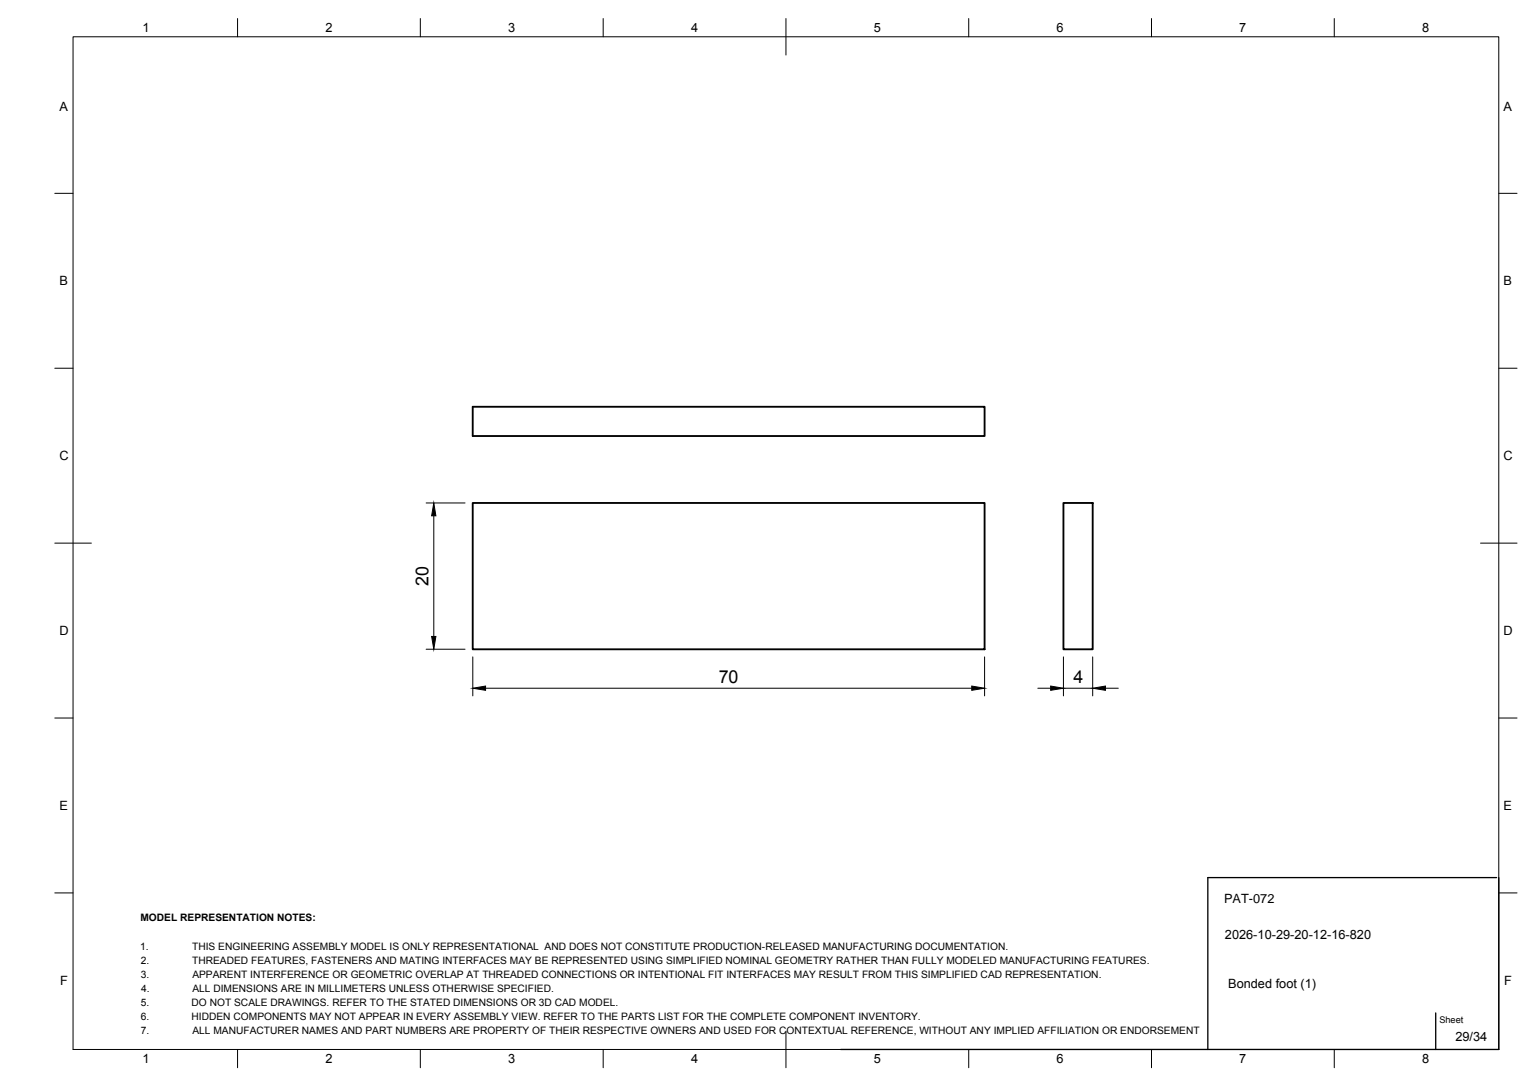
ISO-10303-21;
HEADER;
/* Generated by software containing ST-Developer
 * from STEP Tools, Inc. (www.steptools.com) 
 */

FILE_DESCRIPTION(
/* description */ ('PAT-072'),
/* implementation_level */ '2;1');

FILE_NAME(
/* name */ 'Bonded foot (1).step',
/* time_stamp */ '2026-10-29T20:11:56-07:00',
/* author */ (''),
/* organization */ (''),
/* preprocessor_version */ 'ST-DEVELOPER v20.2',
/* originating_system */ 'Autodesk Translation Framework v15.17.0.0',
/* authorisation */ '');

FILE_SCHEMA (('AUTOMOTIVE_DESIGN { 1 0 10303 214 3 1 1 }'));
ENDSEC;

DATA;
#10=MECHANICAL_DESIGN_GEOMETRIC_PRESENTATION_REPRESENTATION('',(#362),#11432);
#290=SHAPE_REPRESENTATION_RELATIONSHIP('SRR','None',#11594,#326);
#326=ADVANCED_BREP_SHAPE_REPRESENTATION('',(#398),#11425);
#362=STYLED_ITEM('',(#11833),#398);
#398=MANIFOLD_SOLID_BREP('Body1',#6097);
#743=PLANE('',#7087);
#744=PLANE('',#7088);
#745=PLANE('',#7089);
#746=PLANE('',#7090);
#747=PLANE('',#7091);
#748=PLANE('',#7092);
#1091=FACE_OUTER_BOUND('',#1616,.T.);
#1092=FACE_OUTER_BOUND('',#1617,.T.);
#1093=FACE_OUTER_BOUND('',#1618,.T.);
#1094=FACE_OUTER_BOUND('',#1619,.T.);
#1095=FACE_OUTER_BOUND('',#1620,.T.);
#1096=FACE_OUTER_BOUND('',#1621,.T.);
#1616=EDGE_LOOP('',(#5264,#5265,#5266,#5267));
#1617=EDGE_LOOP('',(#5268,#5269,#5270,#5271));
#1618=EDGE_LOOP('',(#5272,#5273,#5274,#5275));
#1619=EDGE_LOOP('',(#5276,#5277,#5278,#5279));
#1620=EDGE_LOOP('',(#5280,#5281,#5282,#5283));
#1621=EDGE_LOOP('',(#5284,#5285,#5286,#5287));
#2019=LINE('',#10983,#2438);
#2020=LINE('',#10985,#2439);
#2021=LINE('',#10987,#2440);
#2022=LINE('',#10988,#2441);
#2023=LINE('',#10991,#2442);
#2024=LINE('',#10993,#2443);
#2025=LINE('',#10994,#2444);
#2026=LINE('',#10997,#2445);
#2027=LINE('',#10999,#2446);
#2028=LINE('',#11000,#2447);
#2029=LINE('',#11002,#2448);
#2030=LINE('',#11003,#2449);
#2438=VECTOR('',#8742,1.);
#2439=VECTOR('',#8743,1.);
#2440=VECTOR('',#8744,1.);
#2441=VECTOR('',#8745,1.);
#2442=VECTOR('',#8748,1.);
#2443=VECTOR('',#8749,1.);
#2444=VECTOR('',#8750,1.);
#2445=VECTOR('',#8753,1.);
#2446=VECTOR('',#8754,1.);
#2447=VECTOR('',#8755,1.);
#2448=VECTOR('',#8758,1.);
#2449=VECTOR('',#8759,1.);
#3228=VERTEX_POINT('',#10981);
#3229=VERTEX_POINT('',#10982);
#3230=VERTEX_POINT('',#10984);
#3231=VERTEX_POINT('',#10986);
#3232=VERTEX_POINT('',#10990);
#3233=VERTEX_POINT('',#10992);
#3234=VERTEX_POINT('',#10996);
#3235=VERTEX_POINT('',#10998);
#3921=EDGE_CURVE('',#3228,#3229,#2019,.T.);
#3922=EDGE_CURVE('',#3229,#3230,#2020,.T.);
#3923=EDGE_CURVE('',#3231,#3230,#2021,.T.);
#3924=EDGE_CURVE('',#3228,#3231,#2022,.T.);
#3925=EDGE_CURVE('',#3232,#3228,#2023,.T.);
#3926=EDGE_CURVE('',#3233,#3231,#2024,.T.);
#3927=EDGE_CURVE('',#3232,#3233,#2025,.T.);
#3928=EDGE_CURVE('',#3234,#3232,#2026,.T.);
#3929=EDGE_CURVE('',#3235,#3233,#2027,.T.);
#3930=EDGE_CURVE('',#3234,#3235,#2028,.T.);
#3931=EDGE_CURVE('',#3229,#3234,#2029,.T.);
#3932=EDGE_CURVE('',#3230,#3235,#2030,.T.);
#5264=ORIENTED_EDGE('',*,*,#3921,.T.);
#5265=ORIENTED_EDGE('',*,*,#3922,.T.);
#5266=ORIENTED_EDGE('',*,*,#3923,.F.);
#5267=ORIENTED_EDGE('',*,*,#3924,.F.);
#5268=ORIENTED_EDGE('',*,*,#3925,.T.);
#5269=ORIENTED_EDGE('',*,*,#3924,.T.);
#5270=ORIENTED_EDGE('',*,*,#3926,.F.);
#5271=ORIENTED_EDGE('',*,*,#3927,.F.);
#5272=ORIENTED_EDGE('',*,*,#3928,.T.);
#5273=ORIENTED_EDGE('',*,*,#3927,.T.);
#5274=ORIENTED_EDGE('',*,*,#3929,.F.);
#5275=ORIENTED_EDGE('',*,*,#3930,.F.);
#5276=ORIENTED_EDGE('',*,*,#3931,.T.);
#5277=ORIENTED_EDGE('',*,*,#3930,.T.);
#5278=ORIENTED_EDGE('',*,*,#3932,.F.);
#5279=ORIENTED_EDGE('',*,*,#3922,.F.);
#5280=ORIENTED_EDGE('',*,*,#3932,.T.);
#5281=ORIENTED_EDGE('',*,*,#3929,.T.);
#5282=ORIENTED_EDGE('',*,*,#3926,.T.);
#5283=ORIENTED_EDGE('',*,*,#3923,.T.);
#5284=ORIENTED_EDGE('',*,*,#3931,.F.);
#5285=ORIENTED_EDGE('',*,*,#3921,.F.);
#5286=ORIENTED_EDGE('',*,*,#3925,.F.);
#5287=ORIENTED_EDGE('',*,*,#3928,.F.);
#5990=ADVANCED_FACE('',(#1091),#743,.T.);
#5991=ADVANCED_FACE('',(#1092),#744,.T.);
#5992=ADVANCED_FACE('',(#1093),#745,.T.);
#5993=ADVANCED_FACE('',(#1094),#746,.T.);
#5994=ADVANCED_FACE('',(#1095),#747,.T.);
#5995=ADVANCED_FACE('',(#1096),#748,.F.);
#6097=CLOSED_SHELL('',(#5990,#5991,#5992,#5993,#5994,#5995));
#7086=AXIS2_PLACEMENT_3D('',#10979,#8738,#8739);
#7087=AXIS2_PLACEMENT_3D('',#10980,#8740,#8741);
#7088=AXIS2_PLACEMENT_3D('',#10989,#8746,#8747);
#7089=AXIS2_PLACEMENT_3D('',#10995,#8751,#8752);
#7090=AXIS2_PLACEMENT_3D('',#11001,#8756,#8757);
#7091=AXIS2_PLACEMENT_3D('',#11004,#8760,#8761);
#7092=AXIS2_PLACEMENT_3D('',#11005,#8762,#8763);
#8738=DIRECTION('axis',(0.,0.,1.));
#8739=DIRECTION('refdir',(1.,0.,0.));
#8740=DIRECTION('center_axis',(0.,1.,0.));
#8741=DIRECTION('ref_axis',(-1.,0.,0.));
#8742=DIRECTION('',(-1.,0.,0.));
#8743=DIRECTION('',(0.,0.,1.));
#8744=DIRECTION('',(-1.,0.,0.));
#8745=DIRECTION('',(0.,0.,1.));
#8746=DIRECTION('center_axis',(1.,0.,0.));
#8747=DIRECTION('ref_axis',(0.,1.,0.));
#8748=DIRECTION('',(0.,1.,0.));
#8749=DIRECTION('',(0.,1.,0.));
#8750=DIRECTION('',(0.,0.,1.));
#8751=DIRECTION('center_axis',(0.,-1.,0.));
#8752=DIRECTION('ref_axis',(1.,0.,0.));
#8753=DIRECTION('',(1.,0.,0.));
#8754=DIRECTION('',(1.,0.,0.));
#8755=DIRECTION('',(0.,0.,1.));
#8756=DIRECTION('center_axis',(-1.,0.,0.));
#8757=DIRECTION('ref_axis',(0.,-1.,0.));
#8758=DIRECTION('',(0.,-1.,0.));
#8759=DIRECTION('',(0.,-1.,0.));
#8760=DIRECTION('center_axis',(0.,0.,1.));
#8761=DIRECTION('ref_axis',(1.,0.,0.));
#8762=DIRECTION('center_axis',(0.,0.,1.));
#8763=DIRECTION('ref_axis',(1.,0.,0.));
#10979=CARTESIAN_POINT('',(0.,0.,0.));
#10980=CARTESIAN_POINT('Origin',(7.,3.5,-0.4));
#10981=CARTESIAN_POINT('',(7.,3.5,-0.4));
#10982=CARTESIAN_POINT('',(5.,3.5,-0.4));
#10983=CARTESIAN_POINT('',(7.,3.5,-0.4));
#10984=CARTESIAN_POINT('',(5.,3.5,0.));
#10985=CARTESIAN_POINT('',(5.,3.5,-0.4));
#10986=CARTESIAN_POINT('',(7.,3.5,0.));
#10987=CARTESIAN_POINT('',(7.,3.5,0.));
#10988=CARTESIAN_POINT('',(7.,3.5,-0.4));
#10989=CARTESIAN_POINT('Origin',(7.,-3.5,-0.4));
#10990=CARTESIAN_POINT('',(7.,-3.5,-0.4));
#10991=CARTESIAN_POINT('',(7.,-3.5,-0.4));
#10992=CARTESIAN_POINT('',(7.,-3.5,0.));
#10993=CARTESIAN_POINT('',(7.,-3.5,0.));
#10994=CARTESIAN_POINT('',(7.,-3.5,-0.4));
#10995=CARTESIAN_POINT('Origin',(5.,-3.5,-0.4));
#10996=CARTESIAN_POINT('',(5.,-3.5,-0.4));
#10997=CARTESIAN_POINT('',(5.,-3.5,-0.4));
#10998=CARTESIAN_POINT('',(5.,-3.5,0.));
#10999=CARTESIAN_POINT('',(5.,-3.5,0.));
#11000=CARTESIAN_POINT('',(5.,-3.5,-0.4));
#11001=CARTESIAN_POINT('Origin',(5.,3.5,-0.4));
#11002=CARTESIAN_POINT('',(5.,3.5,-0.4));
#11003=CARTESIAN_POINT('',(5.,3.5,0.));
#11004=CARTESIAN_POINT('Origin',(6.,0.,0.));
#11005=CARTESIAN_POINT('Origin',(6.,0.,-0.4));
#11386=UNCERTAINTY_MEASURE_WITH_UNIT(LENGTH_MEASURE(0.001),#11433,
'DISTANCE_ACCURACY_VALUE',
'Maximum model space distance between geometric entities at asserted c
onnectivities');
#11393=UNCERTAINTY_MEASURE_WITH_UNIT(LENGTH_MEASURE(0.001),#11433,
'DISTANCE_ACCURACY_VALUE',
'Maximum model space distance between geometric entities at asserted c
onnectivities');
#11425=(
GEOMETRIC_REPRESENTATION_CONTEXT(3)
GLOBAL_UNCERTAINTY_ASSIGNED_CONTEXT((#11386))
GLOBAL_UNIT_ASSIGNED_CONTEXT((#11433,#11435,#11436))
REPRESENTATION_CONTEXT('','3D')
);
#11432=(
GEOMETRIC_REPRESENTATION_CONTEXT(3)
GLOBAL_UNCERTAINTY_ASSIGNED_CONTEXT((#11393))
GLOBAL_UNIT_ASSIGNED_CONTEXT((#11433,#11435,#11436))
REPRESENTATION_CONTEXT('','3D')
);
#11433=(
LENGTH_UNIT()
NAMED_UNIT(*)
SI_UNIT(.CENTI.,.METRE.)
);
#11435=(
NAMED_UNIT(*)
PLANE_ANGLE_UNIT()
SI_UNIT($,.RADIAN.)
);
#11436=(
NAMED_UNIT(*)
SI_UNIT($,.STERADIAN.)
SOLID_ANGLE_UNIT()
);
#11468=SHAPE_DEFINITION_REPRESENTATION(#11506,#11594);
#11506=PRODUCT_DEFINITION_SHAPE('',$,#11633);
#11594=SHAPE_REPRESENTATION('',(#7086),#11425);
#11601=PRODUCT_DEFINITION_CONTEXT('part definition',#11717,'design');
#11633=PRODUCT_DEFINITION('Bonded foot (1)','Bonded foot (1)',
#11671,#11601);
#11671=PRODUCT_DEFINITION_FORMATION('',$,#11750);
#11717=APPLICATION_CONTEXT(
'Core Data for Automotive Mechanical Design Process');
#11718=PRODUCT_CONTEXT('part definition',#11717,'mechanical');
#11750=PRODUCT('Bonded foot (1)','Bonded foot (1)',
'Bonded foot (1)',(#11718));
#11827=COLOUR_RGB('Off White',0.89,0.88,0.83);
#11828=FILL_AREA_STYLE_COLOUR('',#11827);
#11829=FILL_AREA_STYLE('',(#11828));
#11830=SURFACE_STYLE_FILL_AREA(#11829);
#11831=SURFACE_SIDE_STYLE('',(#11830));
#11832=SURFACE_STYLE_USAGE(.BOTH.,#11831);
#11833=PRESENTATION_STYLE_ASSIGNMENT((#11832));
ENDSEC;
END-ISO-10303-21;
